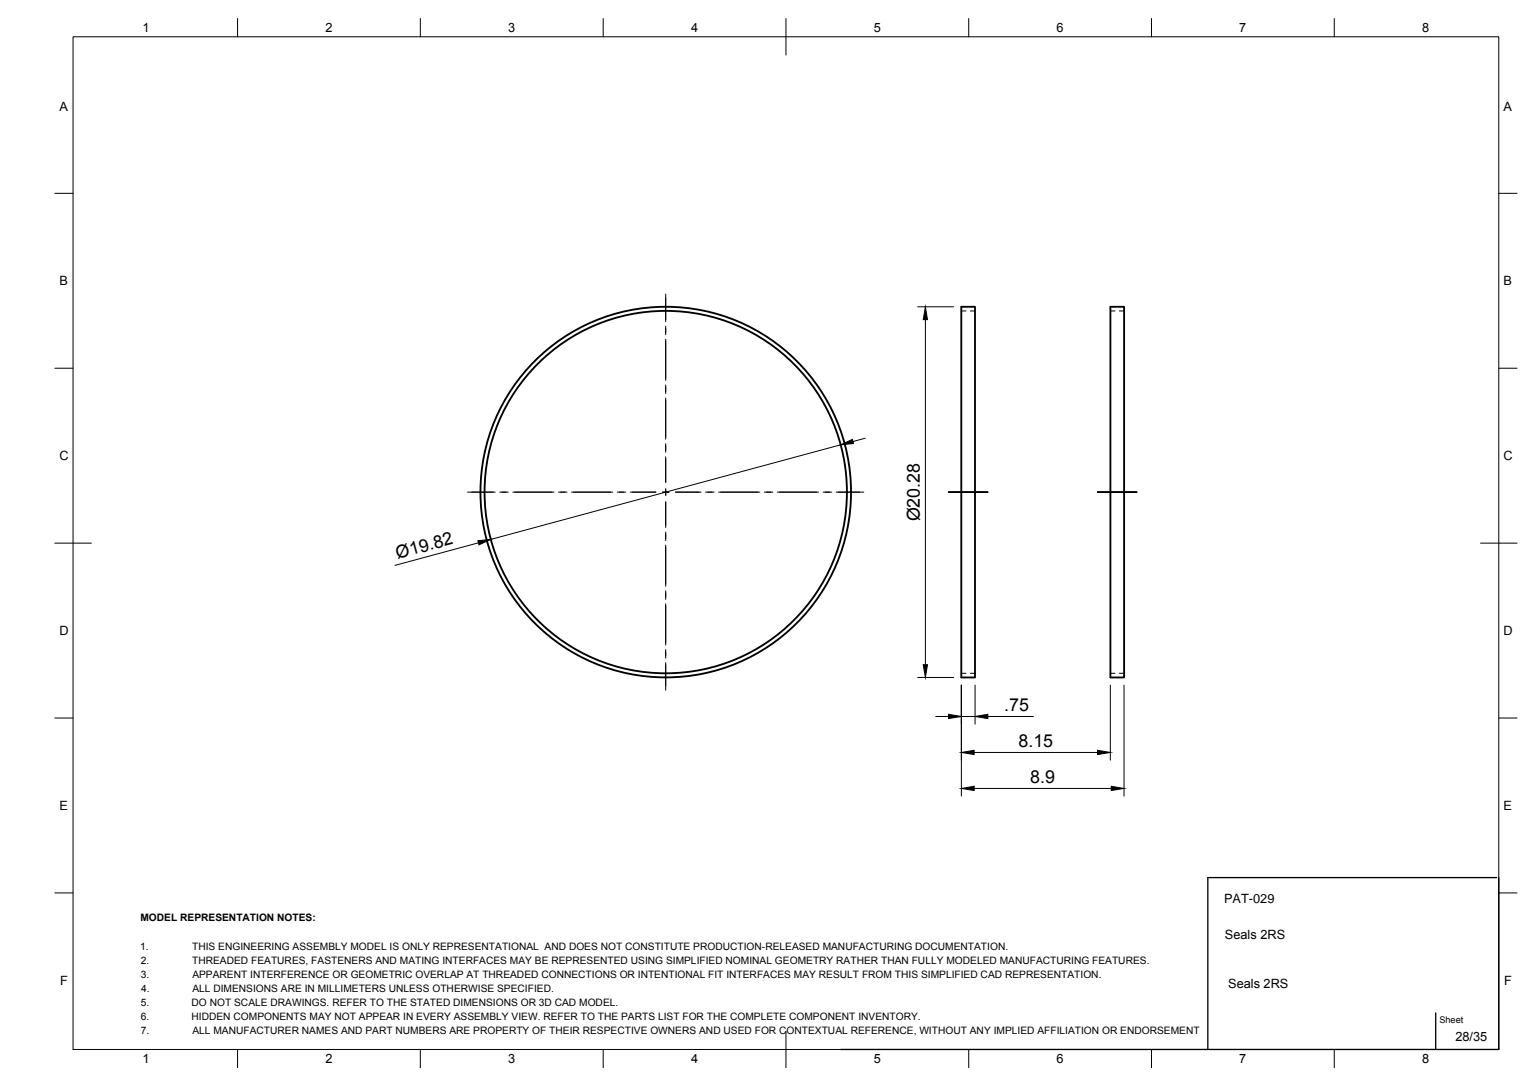
ISO-10303-21;
HEADER;
/* Generated by software containing ST-Developer
 * from STEP Tools, Inc. (www.steptools.com) 
 */

FILE_DESCRIPTION(
/* description */ ('Door-style hinge test fixture with detent'),
/* implementation_level */ '2;1');

FILE_NAME(
/* name */ 'Seals 2RS.step',
/* time_stamp */ '2026-10-28T03:24:57-07:00',
/* author */ (''),
/* organization */ (''),
/* preprocessor_version */ 'ST-DEVELOPER v20.2',
/* originating_system */ 'Autodesk Translation Framework v15.17.0.0',
/* authorisation */ '');

FILE_SCHEMA (('AUTOMOTIVE_DESIGN { 1 0 10303 214 3 1 1 }'));
ENDSEC;

DATA;
#10=MECHANICAL_DESIGN_GEOMETRIC_PRESENTATION_REPRESENTATION('',(#353,#354),#9813);
#283=SHAPE_REPRESENTATION_RELATIONSHIP('SRR','None',#9961,#314);
#314=ADVANCED_BREP_SHAPE_REPRESENTATION('',(#392,#393),#9804);
#353=STYLED_ITEM('',(#10183),#392);
#354=STYLED_ITEM('',(#10183),#393);
#392=MANIFOLD_SOLID_BREP('Body1',#4785);
#393=MANIFOLD_SOLID_BREP('Body2',#4786);
#473=FACE_BOUND('',#1228,.T.);
#474=FACE_BOUND('',#1231,.T.);
#475=FACE_BOUND('',#1234,.T.);
#476=FACE_BOUND('',#1237,.T.);
#618=PLANE('',#5555);
#619=PLANE('',#5560);
#620=PLANE('',#5563);
#621=PLANE('',#5568);
#868=FACE_OUTER_BOUND('',#1227,.T.);
#869=FACE_OUTER_BOUND('',#1229,.T.);
#870=FACE_OUTER_BOUND('',#1230,.T.);
#871=FACE_OUTER_BOUND('',#1232,.T.);
#872=FACE_OUTER_BOUND('',#1233,.T.);
#873=FACE_OUTER_BOUND('',#1235,.T.);
#874=FACE_OUTER_BOUND('',#1236,.T.);
#875=FACE_OUTER_BOUND('',#1238,.T.);
#1227=EDGE_LOOP('',(#4087));
#1228=EDGE_LOOP('',(#4088));
#1229=EDGE_LOOP('',(#4089,#4090,#4091,#4092));
#1230=EDGE_LOOP('',(#4093));
#1231=EDGE_LOOP('',(#4094));
#1232=EDGE_LOOP('',(#4095,#4096,#4097,#4098));
#1233=EDGE_LOOP('',(#4099));
#1234=EDGE_LOOP('',(#4100));
#1235=EDGE_LOOP('',(#4101,#4102,#4103,#4104));
#1236=EDGE_LOOP('',(#4105));
#1237=EDGE_LOOP('',(#4106));
#1238=EDGE_LOOP('',(#4107,#4108,#4109,#4110));
#1569=LINE('',#9331,#1889);
#1570=LINE('',#9336,#1890);
#1571=LINE('',#9345,#1891);
#1572=LINE('',#9350,#1892);
#1889=VECTOR('',#6830,1.013815);
#1890=VECTOR('',#6837,0.991185);
#1891=VECTOR('',#6848,1.013815);
#1892=VECTOR('',#6855,0.991185);
#2160=CIRCLE('',#5556,1.013815);
#2161=CIRCLE('',#5557,0.991185);
#2162=CIRCLE('',#5559,1.013815);
#2163=CIRCLE('',#5561,0.991185);
#2164=CIRCLE('',#5564,1.013815);
#2165=CIRCLE('',#5565,0.991185);
#2166=CIRCLE('',#5567,1.013815);
#2167=CIRCLE('',#5569,0.991185);
#2524=VERTEX_POINT('',#9324);
#2525=VERTEX_POINT('',#9326);
#2526=VERTEX_POINT('',#9329);
#2527=VERTEX_POINT('',#9333);
#2528=VERTEX_POINT('',#9338);
#2529=VERTEX_POINT('',#9340);
#2530=VERTEX_POINT('',#9343);
#2531=VERTEX_POINT('',#9347);
#3060=EDGE_CURVE('',#2524,#2524,#2160,.T.);
#3061=EDGE_CURVE('',#2525,#2525,#2161,.T.);
#3062=EDGE_CURVE('',#2526,#2526,#2162,.T.);
#3063=EDGE_CURVE('',#2526,#2524,#1569,.T.);
#3064=EDGE_CURVE('',#2527,#2527,#2163,.T.);
#3065=EDGE_CURVE('',#2527,#2525,#1570,.T.);
#3066=EDGE_CURVE('',#2528,#2528,#2164,.T.);
#3067=EDGE_CURVE('',#2529,#2529,#2165,.T.);
#3068=EDGE_CURVE('',#2530,#2530,#2166,.T.);
#3069=EDGE_CURVE('',#2530,#2528,#1571,.T.);
#3070=EDGE_CURVE('',#2531,#2531,#2167,.T.);
#3071=EDGE_CURVE('',#2531,#2529,#1572,.T.);
#4087=ORIENTED_EDGE('',*,*,#3060,.F.);
#4088=ORIENTED_EDGE('',*,*,#3061,.T.);
#4089=ORIENTED_EDGE('',*,*,#3062,.F.);
#4090=ORIENTED_EDGE('',*,*,#3063,.T.);
#4091=ORIENTED_EDGE('',*,*,#3060,.T.);
#4092=ORIENTED_EDGE('',*,*,#3063,.F.);
#4093=ORIENTED_EDGE('',*,*,#3062,.T.);
#4094=ORIENTED_EDGE('',*,*,#3064,.F.);
#4095=ORIENTED_EDGE('',*,*,#3064,.T.);
#4096=ORIENTED_EDGE('',*,*,#3065,.T.);
#4097=ORIENTED_EDGE('',*,*,#3061,.F.);
#4098=ORIENTED_EDGE('',*,*,#3065,.F.);
#4099=ORIENTED_EDGE('',*,*,#3066,.F.);
#4100=ORIENTED_EDGE('',*,*,#3067,.T.);
#4101=ORIENTED_EDGE('',*,*,#3068,.F.);
#4102=ORIENTED_EDGE('',*,*,#3069,.T.);
#4103=ORIENTED_EDGE('',*,*,#3066,.T.);
#4104=ORIENTED_EDGE('',*,*,#3069,.F.);
#4105=ORIENTED_EDGE('',*,*,#3068,.T.);
#4106=ORIENTED_EDGE('',*,*,#3070,.F.);
#4107=ORIENTED_EDGE('',*,*,#3070,.T.);
#4108=ORIENTED_EDGE('',*,*,#3071,.T.);
#4109=ORIENTED_EDGE('',*,*,#3067,.F.);
#4110=ORIENTED_EDGE('',*,*,#3071,.F.);
#4441=CYLINDRICAL_SURFACE('',#5558,1.013815);
#4442=CYLINDRICAL_SURFACE('',#5562,0.991185);
#4443=CYLINDRICAL_SURFACE('',#5566,1.013815);
#4444=CYLINDRICAL_SURFACE('',#5570,0.991185);
#4673=ADVANCED_FACE('',(#868,#473),#618,.T.);
#4674=ADVANCED_FACE('',(#869),#4441,.T.);
#4675=ADVANCED_FACE('',(#870,#474),#619,.T.);
#4676=ADVANCED_FACE('',(#871),#4442,.F.);
#4677=ADVANCED_FACE('',(#872,#475),#620,.T.);
#4678=ADVANCED_FACE('',(#873),#4443,.T.);
#4679=ADVANCED_FACE('',(#874,#476),#621,.T.);
#4680=ADVANCED_FACE('',(#875),#4444,.F.);
#4785=CLOSED_SHELL('',(#4673,#4674,#4675,#4676));
#4786=CLOSED_SHELL('',(#4677,#4678,#4679,#4680));
#5554=AXIS2_PLACEMENT_3D('',#9322,#6818,#6819);
#5555=AXIS2_PLACEMENT_3D('',#9323,#6820,#6821);
#5556=AXIS2_PLACEMENT_3D('',#9325,#6822,#6823);
#5557=AXIS2_PLACEMENT_3D('',#9327,#6824,#6825);
#5558=AXIS2_PLACEMENT_3D('',#9328,#6826,#6827);
#5559=AXIS2_PLACEMENT_3D('',#9330,#6828,#6829);
#5560=AXIS2_PLACEMENT_3D('',#9332,#6831,#6832);
#5561=AXIS2_PLACEMENT_3D('',#9334,#6833,#6834);
#5562=AXIS2_PLACEMENT_3D('',#9335,#6835,#6836);
#5563=AXIS2_PLACEMENT_3D('',#9337,#6838,#6839);
#5564=AXIS2_PLACEMENT_3D('',#9339,#6840,#6841);
#5565=AXIS2_PLACEMENT_3D('',#9341,#6842,#6843);
#5566=AXIS2_PLACEMENT_3D('',#9342,#6844,#6845);
#5567=AXIS2_PLACEMENT_3D('',#9344,#6846,#6847);
#5568=AXIS2_PLACEMENT_3D('',#9346,#6849,#6850);
#5569=AXIS2_PLACEMENT_3D('',#9348,#6851,#6852);
#5570=AXIS2_PLACEMENT_3D('',#9349,#6853,#6854);
#6818=DIRECTION('axis',(0.,0.,1.));
#6819=DIRECTION('refdir',(1.,0.,0.));
#6820=DIRECTION('center_axis',(0.,1.,0.));
#6821=DIRECTION('ref_axis',(0.,0.,1.));
#6822=DIRECTION('center_axis',(0.,-1.,0.));
#6823=DIRECTION('ref_axis',(1.,0.,0.));
#6824=DIRECTION('center_axis',(0.,-1.,0.));
#6825=DIRECTION('ref_axis',(1.,0.,0.));
#6826=DIRECTION('center_axis',(0.,-1.,0.));
#6827=DIRECTION('ref_axis',(1.,0.,0.));
#6828=DIRECTION('center_axis',(0.,-1.,0.));
#6829=DIRECTION('ref_axis',(1.,0.,0.));
#6830=DIRECTION('',(0.,1.,0.));
#6831=DIRECTION('center_axis',(0.,-1.,0.));
#6832=DIRECTION('ref_axis',(0.,0.,-1.));
#6833=DIRECTION('center_axis',(0.,-1.,0.));
#6834=DIRECTION('ref_axis',(1.,0.,0.));
#6835=DIRECTION('center_axis',(0.,-1.,0.));
#6836=DIRECTION('ref_axis',(1.,0.,0.));
#6837=DIRECTION('',(0.,1.,0.));
#6838=DIRECTION('center_axis',(0.,1.,0.));
#6839=DIRECTION('ref_axis',(0.,0.,1.));
#6840=DIRECTION('center_axis',(0.,-1.,0.));
#6841=DIRECTION('ref_axis',(1.,0.,0.));
#6842=DIRECTION('center_axis',(0.,-1.,0.));
#6843=DIRECTION('ref_axis',(1.,0.,0.));
#6844=DIRECTION('center_axis',(0.,-1.,0.));
#6845=DIRECTION('ref_axis',(1.,0.,0.));
#6846=DIRECTION('center_axis',(0.,-1.,0.));
#6847=DIRECTION('ref_axis',(1.,0.,0.));
#6848=DIRECTION('',(0.,1.,0.));
#6849=DIRECTION('center_axis',(0.,-1.,0.));
#6850=DIRECTION('ref_axis',(0.,0.,-1.));
#6851=DIRECTION('center_axis',(0.,-1.,0.));
#6852=DIRECTION('ref_axis',(1.,0.,0.));
#6853=DIRECTION('center_axis',(0.,-1.,0.));
#6854=DIRECTION('ref_axis',(1.,0.,0.));
#6855=DIRECTION('',(0.,1.,0.));
#9322=CARTESIAN_POINT('',(0.,0.,0.));
#9323=CARTESIAN_POINT('Origin',(1.013815,0.445,0.));
#9324=CARTESIAN_POINT('',(-1.013815,0.445,-1.24156529467757E-16));
#9325=CARTESIAN_POINT('Origin',(0.,0.445,0.));
#9326=CARTESIAN_POINT('',(-0.991185,0.445,-1.21385153761287E-16));
#9327=CARTESIAN_POINT('Origin',(0.,0.445,0.));
#9328=CARTESIAN_POINT('Origin',(0.,0.4075,0.));
#9329=CARTESIAN_POINT('',(-1.013815,0.37,-1.24156529467757E-16));
#9330=CARTESIAN_POINT('Origin',(0.,0.37,0.));
#9331=CARTESIAN_POINT('',(-1.013815,0.4075,-1.24156529467757E-16));
#9332=CARTESIAN_POINT('Origin',(0.991185,0.37,0.));
#9333=CARTESIAN_POINT('',(-0.991185,0.37,-1.21385153761287E-16));
#9334=CARTESIAN_POINT('Origin',(0.,0.37,0.));
#9335=CARTESIAN_POINT('Origin',(0.,0.4075,0.));
#9336=CARTESIAN_POINT('',(-0.991185,0.4075,-1.21385153761287E-16));
#9337=CARTESIAN_POINT('Origin',(1.013815,-0.37,0.));
#9338=CARTESIAN_POINT('',(-1.013815,-0.37,-1.24156529467757E-16));
#9339=CARTESIAN_POINT('Origin',(0.,-0.37,0.));
#9340=CARTESIAN_POINT('',(-0.991185,-0.37,-1.21385153761287E-16));
#9341=CARTESIAN_POINT('Origin',(0.,-0.37,0.));
#9342=CARTESIAN_POINT('Origin',(0.,-0.4075,0.));
#9343=CARTESIAN_POINT('',(-1.013815,-0.445,-1.24156529467757E-16));
#9344=CARTESIAN_POINT('Origin',(0.,-0.445,0.));
#9345=CARTESIAN_POINT('',(-1.013815,-0.4075,-1.24156529467757E-16));
#9346=CARTESIAN_POINT('Origin',(0.991185,-0.445,0.));
#9347=CARTESIAN_POINT('',(-0.991185,-0.445,-1.21385153761287E-16));
#9348=CARTESIAN_POINT('Origin',(0.,-0.445,0.));
#9349=CARTESIAN_POINT('Origin',(0.,-0.4075,0.));
#9350=CARTESIAN_POINT('',(-0.991185,-0.4075,-1.21385153761287E-16));
#9768=UNCERTAINTY_MEASURE_WITH_UNIT(LENGTH_MEASURE(0.001),#9814,
'DISTANCE_ACCURACY_VALUE',
'Maximum model space distance between geometric entities at asserted c
onnectivities');
#9777=UNCERTAINTY_MEASURE_WITH_UNIT(LENGTH_MEASURE(0.001),#9814,
'DISTANCE_ACCURACY_VALUE',
'Maximum model space distance between geometric entities at asserted c
onnectivities');
#9804=(
GEOMETRIC_REPRESENTATION_CONTEXT(3)
GLOBAL_UNCERTAINTY_ASSIGNED_CONTEXT((#9768))
GLOBAL_UNIT_ASSIGNED_CONTEXT((#9814,#9816,#9817))
REPRESENTATION_CONTEXT('','3D')
);
#9813=(
GEOMETRIC_REPRESENTATION_CONTEXT(3)
GLOBAL_UNCERTAINTY_ASSIGNED_CONTEXT((#9777))
GLOBAL_UNIT_ASSIGNED_CONTEXT((#9814,#9816,#9817))
REPRESENTATION_CONTEXT('','3D')
);
#9814=(
LENGTH_UNIT()
NAMED_UNIT(*)
SI_UNIT(.CENTI.,.METRE.)
);
#9816=(
NAMED_UNIT(*)
PLANE_ANGLE_UNIT()
SI_UNIT($,.RADIAN.)
);
#9817=(
NAMED_UNIT(*)
SI_UNIT($,.STERADIAN.)
SOLID_ANGLE_UNIT()
);
#9844=SHAPE_DEFINITION_REPRESENTATION(#9879,#9961);
#9879=PRODUCT_DEFINITION_SHAPE('',$,#9997);
#9961=SHAPE_REPRESENTATION('',(#5554),#9804);
#9970=PRODUCT_DEFINITION_CONTEXT('part definition',#10077,'design');
#9997=PRODUCT_DEFINITION('Seals 2RS','Seals 2RS',#10032,#9970);
#10032=PRODUCT_DEFINITION_FORMATION('',$,#10105);
#10077=APPLICATION_CONTEXT(
'Core Data for Automotive Mechanical Design Process');
#10078=PRODUCT_CONTEXT('part definition',#10077,'mechanical');
#10105=PRODUCT('Seals 2RS','Seals 2RS','Seals 2RS',(#10078));
#10177=COLOUR_RGB('Grey',0.48,0.52,0.57);
#10178=FILL_AREA_STYLE_COLOUR('',#10177);
#10179=FILL_AREA_STYLE('',(#10178));
#10180=SURFACE_STYLE_FILL_AREA(#10179);
#10181=SURFACE_SIDE_STYLE('',(#10180));
#10182=SURFACE_STYLE_USAGE(.BOTH.,#10181);
#10183=PRESENTATION_STYLE_ASSIGNMENT((#10182));
ENDSEC;
END-ISO-10303-21;
